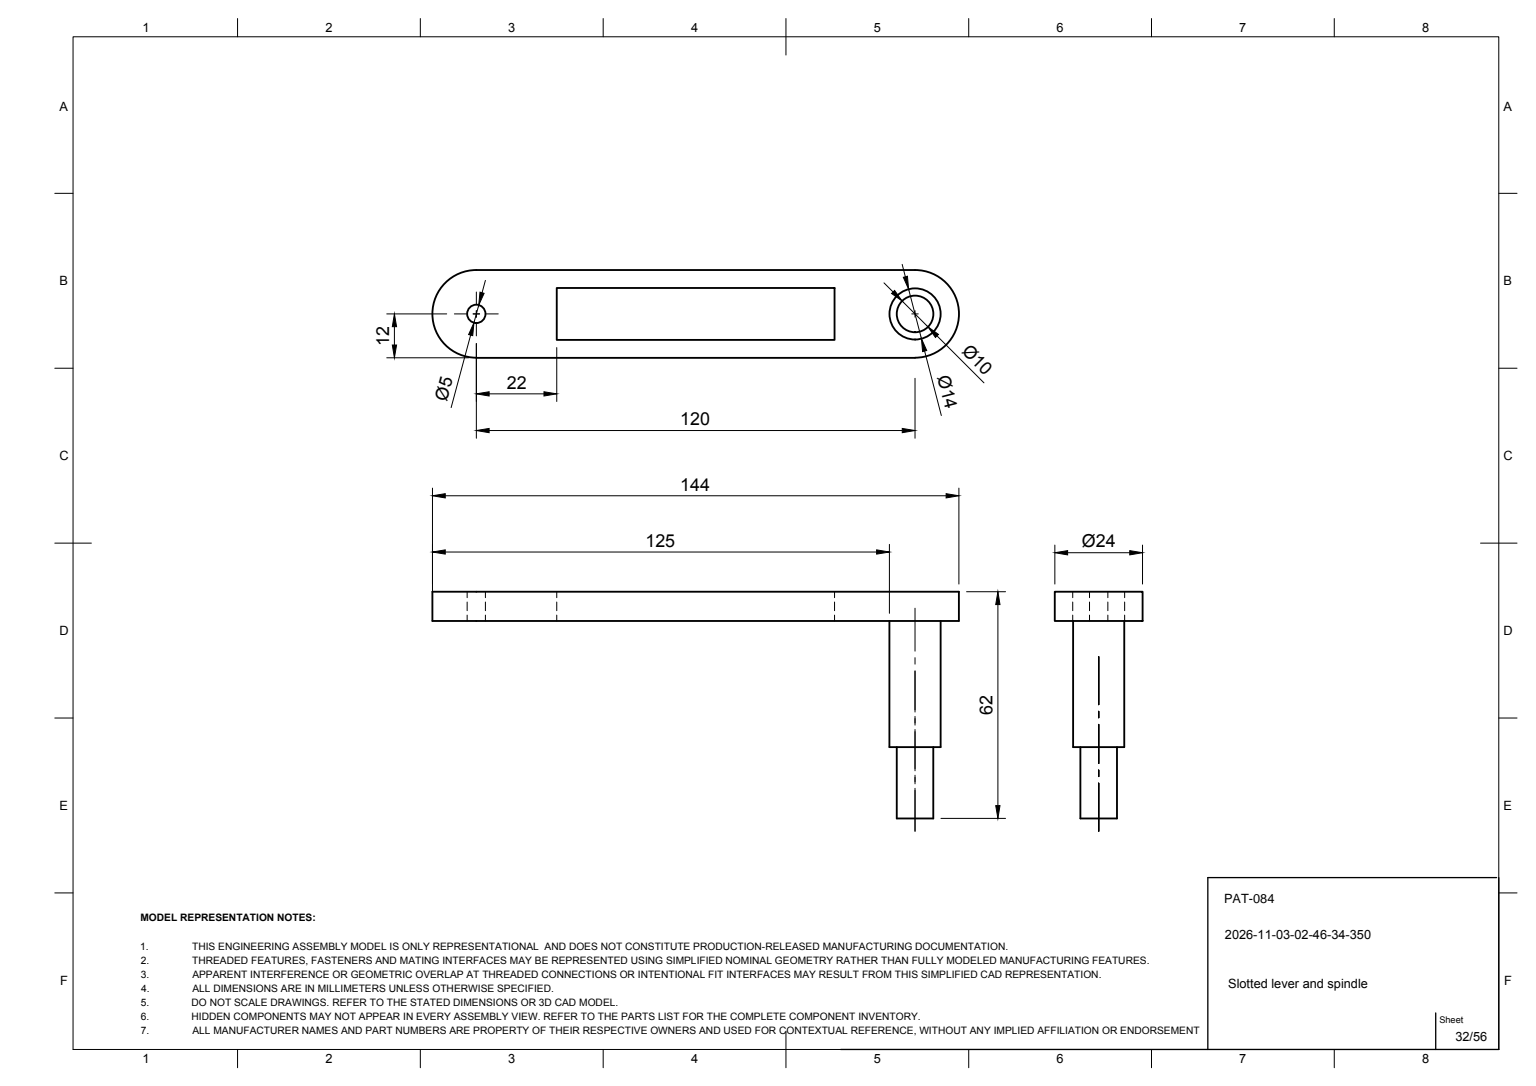
ISO-10303-21;
HEADER;
/* Generated by software containing ST-Developer
 * from STEP Tools, Inc. (www.steptools.com) 
 */

FILE_DESCRIPTION(
/* description */ ('Quick-return (Whitworth) mechanism'),
/* implementation_level */ '2;1');

FILE_NAME(
/* name */ 'Slotted lever and spindle.step',
/* time_stamp */ '2026-10-28T03:25:57-07:00',
/* author */ (''),
/* organization */ (''),
/* preprocessor_version */ 'ST-DEVELOPER v20.2',
/* originating_system */ 'Autodesk Translation Framework v15.17.0.0',
/* authorisation */ '');

FILE_SCHEMA (('AUTOMOTIVE_DESIGN { 1 0 10303 214 3 1 1 }'));
ENDSEC;

DATA;
#10=MECHANICAL_DESIGN_GEOMETRIC_PRESENTATION_REPRESENTATION('',(#520),#14878);
#424=SHAPE_REPRESENTATION_RELATIONSHIP('SRR','None',#15095,#468);
#468=ADVANCED_BREP_SHAPE_REPRESENTATION('',(#571),#14852);
#520=STYLED_ITEM('',(#15399),#571);
#571=MANIFOLD_SOLID_BREP('Body1',#7875);
#725=FACE_BOUND('',#1925,.T.);
#726=FACE_BOUND('',#1926,.T.);
#727=FACE_BOUND('',#1927,.T.);
#728=FACE_BOUND('',#1932,.T.);
#729=FACE_BOUND('',#1936,.T.);
#730=FACE_BOUND('',#1937,.T.);
#912=PLANE('',#8985);
#913=PLANE('',#8986);
#914=PLANE('',#8987);
#915=PLANE('',#8988);
#916=PLANE('',#8992);
#917=PLANE('',#8995);
#918=PLANE('',#8996);
#919=PLANE('',#8999);
#920=PLANE('',#9005);
#921=PLANE('',#9006);
#1318=FACE_OUTER_BOUND('',#1918,.T.);
#1319=FACE_OUTER_BOUND('',#1919,.T.);
#1320=FACE_OUTER_BOUND('',#1920,.T.);
#1321=FACE_OUTER_BOUND('',#1921,.T.);
#1322=FACE_OUTER_BOUND('',#1922,.T.);
#1323=FACE_OUTER_BOUND('',#1923,.T.);
#1324=FACE_OUTER_BOUND('',#1924,.T.);
#1325=FACE_OUTER_BOUND('',#1928,.T.);
#1326=FACE_OUTER_BOUND('',#1929,.T.);
#1327=FACE_OUTER_BOUND('',#1930,.T.);
#1328=FACE_OUTER_BOUND('',#1931,.T.);
#1329=FACE_OUTER_BOUND('',#1933,.T.);
#1330=FACE_OUTER_BOUND('',#1934,.T.);
#1331=FACE_OUTER_BOUND('',#1935,.T.);
#1332=FACE_OUTER_BOUND('',#1938,.T.);
#1918=EDGE_LOOP('',(#6382,#6383,#6384,#6385));
#1919=EDGE_LOOP('',(#6386,#6387,#6388,#6389));
#1920=EDGE_LOOP('',(#6390,#6391,#6392,#6393));
#1921=EDGE_LOOP('',(#6394,#6395,#6396,#6397));
#1922=EDGE_LOOP('',(#6398,#6399,#6400,#6401));
#1923=EDGE_LOOP('',(#6402,#6403,#6404,#6405));
#1924=EDGE_LOOP('',(#6406,#6407,#6408,#6409));
#1925=EDGE_LOOP('',(#6410));
#1926=EDGE_LOOP('',(#6411,#6412,#6413,#6414));
#1927=EDGE_LOOP('',(#6415));
#1928=EDGE_LOOP('',(#6416,#6417,#6418,#6419));
#1929=EDGE_LOOP('',(#6420,#6421,#6422,#6423));
#1930=EDGE_LOOP('',(#6424,#6425,#6426,#6427));
#1931=EDGE_LOOP('',(#6428));
#1932=EDGE_LOOP('',(#6429));
#1933=EDGE_LOOP('',(#6430,#6431,#6432,#6433));
#1934=EDGE_LOOP('',(#6434,#6435,#6436,#6437));
#1935=EDGE_LOOP('',(#6438,#6439,#6440,#6441));
#1936=EDGE_LOOP('',(#6442));
#1937=EDGE_LOOP('',(#6443,#6444,#6445,#6446));
#1938=EDGE_LOOP('',(#6447));
#2405=LINE('',#13732,#2928);
#2406=LINE('',#13737,#2929);
#2407=LINE('',#13739,#2930);
#2408=LINE('',#13741,#2931);
#2409=LINE('',#13742,#2932);
#2410=LINE('',#13745,#2933);
#2411=LINE('',#13747,#2934);
#2412=LINE('',#13748,#2935);
#2413=LINE('',#13751,#2936);
#2414=LINE('',#13753,#2937);
#2415=LINE('',#13754,#2938);
#2416=LINE('',#13756,#2939);
#2417=LINE('',#13757,#2940);
#2418=LINE('',#13761,#2941);
#2419=LINE('',#13765,#2942);
#2420=LINE('',#13769,#2943);
#2421=LINE('',#13772,#2944);
#2422=LINE('',#13777,#2945);
#2423=LINE('',#13778,#2946);
#2424=LINE('',#13781,#2947);
#2425=LINE('',#13782,#2948);
#2426=LINE('',#13791,#2949);
#2427=LINE('',#13794,#2950);
#2928=VECTOR('',#10832,0.25);
#2929=VECTOR('',#10837,1.);
#2930=VECTOR('',#10838,1.);
#2931=VECTOR('',#10839,1.);
#2932=VECTOR('',#10840,1.);
#2933=VECTOR('',#10843,1.);
#2934=VECTOR('',#10844,1.);
#2935=VECTOR('',#10845,1.);
#2936=VECTOR('',#10848,1.);
#2937=VECTOR('',#10849,1.);
#2938=VECTOR('',#10850,1.);
#2939=VECTOR('',#10853,1.);
#2940=VECTOR('',#10854,1.);
#2941=VECTOR('',#10857,1.);
#2942=VECTOR('',#10860,1.);
#2943=VECTOR('',#10865,1.);
#2944=VECTOR('',#10868,1.);
#2945=VECTOR('',#10873,1.);
#2946=VECTOR('',#10874,1.);
#2947=VECTOR('',#10877,1.);
#2948=VECTOR('',#10878,1.);
#2949=VECTOR('',#10891,0.7);
#2950=VECTOR('',#10894,0.5);
#3510=CIRCLE('',#8983,0.25);
#3511=CIRCLE('',#8984,0.25);
#3512=CIRCLE('',#8990,1.2);
#3513=CIRCLE('',#8991,1.2);
#3514=CIRCLE('',#8993,1.2);
#3515=CIRCLE('',#8994,0.7);
#3516=CIRCLE('',#8998,1.2);
#3517=CIRCLE('',#9000,0.7);
#3518=CIRCLE('',#9001,0.5);
#3519=CIRCLE('',#9004,0.5);
#4014=VERTEX_POINT('',#13729);
#4015=VERTEX_POINT('',#13731);
#4016=VERTEX_POINT('',#13735);
#4017=VERTEX_POINT('',#13736);
#4018=VERTEX_POINT('',#13738);
#4019=VERTEX_POINT('',#13740);
#4020=VERTEX_POINT('',#13744);
#4021=VERTEX_POINT('',#13746);
#4022=VERTEX_POINT('',#13750);
#4023=VERTEX_POINT('',#13752);
#4024=VERTEX_POINT('',#13759);
#4025=VERTEX_POINT('',#13760);
#4026=VERTEX_POINT('',#13762);
#4027=VERTEX_POINT('',#13764);
#4028=VERTEX_POINT('',#13768);
#4029=VERTEX_POINT('',#13770);
#4030=VERTEX_POINT('',#13773);
#4031=VERTEX_POINT('',#13776);
#4032=VERTEX_POINT('',#13780);
#4033=VERTEX_POINT('',#13786);
#4034=VERTEX_POINT('',#13788);
#4035=VERTEX_POINT('',#13793);
#4848=EDGE_CURVE('',#4014,#4014,#3510,.T.);
#4849=EDGE_CURVE('',#4014,#4015,#2405,.T.);
#4850=EDGE_CURVE('',#4015,#4015,#3511,.T.);
#4851=EDGE_CURVE('',#4016,#4017,#2406,.T.);
#4852=EDGE_CURVE('',#4016,#4018,#2407,.T.);
#4853=EDGE_CURVE('',#4019,#4018,#2408,.T.);
#4854=EDGE_CURVE('',#4017,#4019,#2409,.T.);
#4855=EDGE_CURVE('',#4017,#4020,#2410,.T.);
#4856=EDGE_CURVE('',#4021,#4019,#2411,.T.);
#4857=EDGE_CURVE('',#4020,#4021,#2412,.T.);
#4858=EDGE_CURVE('',#4020,#4022,#2413,.T.);
#4859=EDGE_CURVE('',#4023,#4021,#2414,.T.);
#4860=EDGE_CURVE('',#4022,#4023,#2415,.T.);
#4861=EDGE_CURVE('',#4022,#4016,#2416,.T.);
#4862=EDGE_CURVE('',#4018,#4023,#2417,.T.);
#4863=EDGE_CURVE('',#4024,#4025,#2418,.T.);
#4864=EDGE_CURVE('',#4026,#4025,#3512,.T.);
#4865=EDGE_CURVE('',#4027,#4026,#2419,.T.);
#4866=EDGE_CURVE('',#4027,#4024,#3513,.T.);
#4867=EDGE_CURVE('',#4027,#4028,#2420,.T.);
#4868=EDGE_CURVE('',#4029,#4028,#3514,.T.);
#4869=EDGE_CURVE('',#4029,#4024,#2421,.T.);
#4870=EDGE_CURVE('',#4030,#4030,#3515,.T.);
#4871=EDGE_CURVE('',#4031,#4029,#2422,.T.);
#4872=EDGE_CURVE('',#4025,#4031,#2423,.T.);
#4873=EDGE_CURVE('',#4032,#4026,#2424,.T.);
#4874=EDGE_CURVE('',#4028,#4032,#2425,.T.);
#4875=EDGE_CURVE('',#4031,#4032,#3516,.T.);
#4876=EDGE_CURVE('',#4033,#4033,#3517,.T.);
#4877=EDGE_CURVE('',#4034,#4034,#3518,.T.);
#4878=EDGE_CURVE('',#4030,#4033,#2426,.T.);
#4879=EDGE_CURVE('',#4034,#4035,#2427,.T.);
#4880=EDGE_CURVE('',#4035,#4035,#3519,.T.);
#6382=ORIENTED_EDGE('',*,*,#4848,.F.);
#6383=ORIENTED_EDGE('',*,*,#4849,.T.);
#6384=ORIENTED_EDGE('',*,*,#4850,.F.);
#6385=ORIENTED_EDGE('',*,*,#4849,.F.);
#6386=ORIENTED_EDGE('',*,*,#4851,.F.);
#6387=ORIENTED_EDGE('',*,*,#4852,.T.);
#6388=ORIENTED_EDGE('',*,*,#4853,.F.);
#6389=ORIENTED_EDGE('',*,*,#4854,.F.);
#6390=ORIENTED_EDGE('',*,*,#4855,.F.);
#6391=ORIENTED_EDGE('',*,*,#4854,.T.);
#6392=ORIENTED_EDGE('',*,*,#4856,.F.);
#6393=ORIENTED_EDGE('',*,*,#4857,.F.);
#6394=ORIENTED_EDGE('',*,*,#4858,.F.);
#6395=ORIENTED_EDGE('',*,*,#4857,.T.);
#6396=ORIENTED_EDGE('',*,*,#4859,.F.);
#6397=ORIENTED_EDGE('',*,*,#4860,.F.);
#6398=ORIENTED_EDGE('',*,*,#4861,.F.);
#6399=ORIENTED_EDGE('',*,*,#4860,.T.);
#6400=ORIENTED_EDGE('',*,*,#4862,.F.);
#6401=ORIENTED_EDGE('',*,*,#4852,.F.);
#6402=ORIENTED_EDGE('',*,*,#4863,.T.);
#6403=ORIENTED_EDGE('',*,*,#4864,.F.);
#6404=ORIENTED_EDGE('',*,*,#4865,.F.);
#6405=ORIENTED_EDGE('',*,*,#4866,.T.);
#6406=ORIENTED_EDGE('',*,*,#4867,.T.);
#6407=ORIENTED_EDGE('',*,*,#4868,.F.);
#6408=ORIENTED_EDGE('',*,*,#4869,.T.);
#6409=ORIENTED_EDGE('',*,*,#4866,.F.);
#6410=ORIENTED_EDGE('',*,*,#4848,.T.);
#6411=ORIENTED_EDGE('',*,*,#4858,.T.);
#6412=ORIENTED_EDGE('',*,*,#4861,.T.);
#6413=ORIENTED_EDGE('',*,*,#4851,.T.);
#6414=ORIENTED_EDGE('',*,*,#4855,.T.);
#6415=ORIENTED_EDGE('',*,*,#4870,.T.);
#6416=ORIENTED_EDGE('',*,*,#4869,.F.);
#6417=ORIENTED_EDGE('',*,*,#4871,.F.);
#6418=ORIENTED_EDGE('',*,*,#4872,.F.);
#6419=ORIENTED_EDGE('',*,*,#4863,.F.);
#6420=ORIENTED_EDGE('',*,*,#4867,.F.);
#6421=ORIENTED_EDGE('',*,*,#4865,.T.);
#6422=ORIENTED_EDGE('',*,*,#4873,.F.);
#6423=ORIENTED_EDGE('',*,*,#4874,.F.);
#6424=ORIENTED_EDGE('',*,*,#4871,.T.);
#6425=ORIENTED_EDGE('',*,*,#4868,.T.);
#6426=ORIENTED_EDGE('',*,*,#4874,.T.);
#6427=ORIENTED_EDGE('',*,*,#4875,.F.);
#6428=ORIENTED_EDGE('',*,*,#4876,.F.);
#6429=ORIENTED_EDGE('',*,*,#4877,.F.);
#6430=ORIENTED_EDGE('',*,*,#4870,.F.);
#6431=ORIENTED_EDGE('',*,*,#4878,.T.);
#6432=ORIENTED_EDGE('',*,*,#4876,.T.);
#6433=ORIENTED_EDGE('',*,*,#4878,.F.);
#6434=ORIENTED_EDGE('',*,*,#4877,.T.);
#6435=ORIENTED_EDGE('',*,*,#4879,.T.);
#6436=ORIENTED_EDGE('',*,*,#4880,.T.);
#6437=ORIENTED_EDGE('',*,*,#4879,.F.);
#6438=ORIENTED_EDGE('',*,*,#4872,.T.);
#6439=ORIENTED_EDGE('',*,*,#4875,.T.);
#6440=ORIENTED_EDGE('',*,*,#4873,.T.);
#6441=ORIENTED_EDGE('',*,*,#4864,.T.);
#6442=ORIENTED_EDGE('',*,*,#4850,.T.);
#6443=ORIENTED_EDGE('',*,*,#4859,.T.);
#6444=ORIENTED_EDGE('',*,*,#4856,.T.);
#6445=ORIENTED_EDGE('',*,*,#4853,.T.);
#6446=ORIENTED_EDGE('',*,*,#4862,.T.);
#6447=ORIENTED_EDGE('',*,*,#4880,.F.);
#7325=CYLINDRICAL_SURFACE('',#8982,0.25);
#7326=CYLINDRICAL_SURFACE('',#8989,1.2);
#7327=CYLINDRICAL_SURFACE('',#8997,1.2);
#7328=CYLINDRICAL_SURFACE('',#9002,0.7);
#7329=CYLINDRICAL_SURFACE('',#9003,0.5);
#7649=ADVANCED_FACE('',(#1318),#7325,.F.);
#7650=ADVANCED_FACE('',(#1319),#912,.F.);
#7651=ADVANCED_FACE('',(#1320),#913,.F.);
#7652=ADVANCED_FACE('',(#1321),#914,.F.);
#7653=ADVANCED_FACE('',(#1322),#915,.F.);
#7654=ADVANCED_FACE('',(#1323),#7326,.T.);
#7655=ADVANCED_FACE('',(#1324,#725,#726,#727),#916,.F.);
#7656=ADVANCED_FACE('',(#1325),#917,.T.);
#7657=ADVANCED_FACE('',(#1326),#918,.T.);
#7658=ADVANCED_FACE('',(#1327),#7327,.T.);
#7659=ADVANCED_FACE('',(#1328,#728),#919,.F.);
#7660=ADVANCED_FACE('',(#1329),#7328,.T.);
#7661=ADVANCED_FACE('',(#1330),#7329,.T.);
#7662=ADVANCED_FACE('',(#1331,#729,#730),#920,.T.);
#7663=ADVANCED_FACE('',(#1332),#921,.F.);
#7875=CLOSED_SHELL('',(#7649,#7650,#7651,#7652,#7653,#7654,#7655,#7656,
#7657,#7658,#7659,#7660,#7661,#7662,#7663));
#8981=AXIS2_PLACEMENT_3D('',#13727,#10826,#10827);
#8982=AXIS2_PLACEMENT_3D('',#13728,#10828,#10829);
#8983=AXIS2_PLACEMENT_3D('',#13730,#10830,#10831);
#8984=AXIS2_PLACEMENT_3D('',#13733,#10833,#10834);
#8985=AXIS2_PLACEMENT_3D('',#13734,#10835,#10836);
#8986=AXIS2_PLACEMENT_3D('',#13743,#10841,#10842);
#8987=AXIS2_PLACEMENT_3D('',#13749,#10846,#10847);
#8988=AXIS2_PLACEMENT_3D('',#13755,#10851,#10852);
#8989=AXIS2_PLACEMENT_3D('',#13758,#10855,#10856);
#8990=AXIS2_PLACEMENT_3D('',#13763,#10858,#10859);
#8991=AXIS2_PLACEMENT_3D('',#13766,#10861,#10862);
#8992=AXIS2_PLACEMENT_3D('',#13767,#10863,#10864);
#8993=AXIS2_PLACEMENT_3D('',#13771,#10866,#10867);
#8994=AXIS2_PLACEMENT_3D('',#13774,#10869,#10870);
#8995=AXIS2_PLACEMENT_3D('',#13775,#10871,#10872);
#8996=AXIS2_PLACEMENT_3D('',#13779,#10875,#10876);
#8997=AXIS2_PLACEMENT_3D('',#13783,#10879,#10880);
#8998=AXIS2_PLACEMENT_3D('',#13784,#10881,#10882);
#8999=AXIS2_PLACEMENT_3D('',#13785,#10883,#10884);
#9000=AXIS2_PLACEMENT_3D('',#13787,#10885,#10886);
#9001=AXIS2_PLACEMENT_3D('',#13789,#10887,#10888);
#9002=AXIS2_PLACEMENT_3D('',#13790,#10889,#10890);
#9003=AXIS2_PLACEMENT_3D('',#13792,#10892,#10893);
#9004=AXIS2_PLACEMENT_3D('',#13795,#10895,#10896);
#9005=AXIS2_PLACEMENT_3D('',#13796,#10897,#10898);
#9006=AXIS2_PLACEMENT_3D('',#13797,#10899,#10900);
#10826=DIRECTION('axis',(0.,0.,1.));
#10827=DIRECTION('refdir',(1.,0.,0.));
#10828=DIRECTION('center_axis',(0.,0.,1.));
#10829=DIRECTION('ref_axis',(1.,0.,0.));
#10830=DIRECTION('center_axis',(0.,0.,1.));
#10831=DIRECTION('ref_axis',(1.,0.,0.));
#10832=DIRECTION('',(0.,0.,1.));
#10833=DIRECTION('center_axis',(0.,0.,-1.));
#10834=DIRECTION('ref_axis',(1.,0.,0.));
#10835=DIRECTION('center_axis',(0.,-1.,0.));
#10836=DIRECTION('ref_axis',(1.,0.,0.));
#10837=DIRECTION('',(1.,0.,0.));
#10838=DIRECTION('',(0.,0.,1.));
#10839=DIRECTION('',(-1.,0.,0.));
#10840=DIRECTION('',(0.,0.,1.));
#10841=DIRECTION('center_axis',(1.,0.,0.));
#10842=DIRECTION('ref_axis',(0.,1.,0.));
#10843=DIRECTION('',(0.,1.,0.));
#10844=DIRECTION('',(0.,-1.,0.));
#10845=DIRECTION('',(0.,0.,1.));
#10846=DIRECTION('center_axis',(0.,1.,0.));
#10847=DIRECTION('ref_axis',(-1.,0.,0.));
#10848=DIRECTION('',(-1.,0.,0.));
#10849=DIRECTION('',(1.,0.,0.));
#10850=DIRECTION('',(0.,0.,1.));
#10851=DIRECTION('center_axis',(-1.,0.,0.));
#10852=DIRECTION('ref_axis',(0.,-1.,0.));
#10853=DIRECTION('',(0.,-1.,0.));
#10854=DIRECTION('',(0.,1.,0.));
#10855=DIRECTION('center_axis',(0.,0.,1.));
#10856=DIRECTION('ref_axis',(1.,0.,0.));
#10857=DIRECTION('',(0.,0.,1.));
#10858=DIRECTION('center_axis',(0.,0.,1.));
#10859=DIRECTION('ref_axis',(1.,0.,0.));
#10860=DIRECTION('',(0.,0.,1.));
#10861=DIRECTION('center_axis',(0.,0.,1.));
#10862=DIRECTION('ref_axis',(1.,0.,0.));
#10863=DIRECTION('center_axis',(0.,0.,1.));
#10864=DIRECTION('ref_axis',(1.,0.,0.));
#10865=DIRECTION('',(0.,-1.,0.));
#10866=DIRECTION('center_axis',(0.,0.,1.));
#10867=DIRECTION('ref_axis',(1.,0.,0.));
#10868=DIRECTION('',(0.,1.,0.));
#10869=DIRECTION('center_axis',(0.,0.,1.));
#10870=DIRECTION('ref_axis',(1.,0.,0.));
#10871=DIRECTION('center_axis',(-1.,0.,0.));
#10872=DIRECTION('ref_axis',(0.,-1.,0.));
#10873=DIRECTION('',(0.,0.,-1.));
#10874=DIRECTION('',(0.,-1.,0.));
#10875=DIRECTION('center_axis',(1.,0.,0.));
#10876=DIRECTION('ref_axis',(0.,1.,0.));
#10877=DIRECTION('',(0.,1.,0.));
#10878=DIRECTION('',(0.,0.,1.));
#10879=DIRECTION('center_axis',(0.,0.,1.));
#10880=DIRECTION('ref_axis',(1.,0.,0.));
#10881=DIRECTION('center_axis',(0.,0.,1.));
#10882=DIRECTION('ref_axis',(1.,0.,0.));
#10883=DIRECTION('center_axis',(0.,0.,1.));
#10884=DIRECTION('ref_axis',(1.,0.,0.));
#10885=DIRECTION('center_axis',(0.,0.,1.));
#10886=DIRECTION('ref_axis',(1.,0.,0.));
#10887=DIRECTION('center_axis',(0.,0.,-1.));
#10888=DIRECTION('ref_axis',(1.,0.,0.));
#10889=DIRECTION('center_axis',(0.,0.,1.));
#10890=DIRECTION('ref_axis',(1.,0.,0.));
#10891=DIRECTION('',(0.,0.,-1.));
#10892=DIRECTION('center_axis',(0.,0.,1.));
#10893=DIRECTION('ref_axis',(1.,0.,0.));
#10894=DIRECTION('',(0.,0.,-1.));
#10895=DIRECTION('center_axis',(0.,0.,1.));
#10896=DIRECTION('ref_axis',(1.,0.,0.));
#10897=DIRECTION('center_axis',(0.,0.,1.));
#10898=DIRECTION('ref_axis',(1.,0.,0.));
#10899=DIRECTION('center_axis',(0.,0.,1.));
#10900=DIRECTION('ref_axis',(1.,0.,0.));
#13727=CARTESIAN_POINT('',(0.,0.,0.));
#13728=CARTESIAN_POINT('Origin',(0.,12.,6.3));
#13729=CARTESIAN_POINT('',(-0.25,12.,6.4));
#13730=CARTESIAN_POINT('Origin',(0.,12.,6.4));
#13731=CARTESIAN_POINT('',(-0.25,12.,7.2));
#13732=CARTESIAN_POINT('',(-0.25,12.,6.3));
#13733=CARTESIAN_POINT('Origin',(0.,12.,7.2));
#13734=CARTESIAN_POINT('Origin',(-0.71,2.2,6.3));
#13735=CARTESIAN_POINT('',(-0.71,2.2,6.4));
#13736=CARTESIAN_POINT('',(0.71,2.2,6.4));
#13737=CARTESIAN_POINT('',(-0.355,2.2,6.4));
#13738=CARTESIAN_POINT('',(-0.71,2.2,7.2));
#13739=CARTESIAN_POINT('',(-0.71,2.2,6.3));
#13740=CARTESIAN_POINT('',(0.71,2.2,7.2));
#13741=CARTESIAN_POINT('',(-0.355,2.2,7.2));
#13742=CARTESIAN_POINT('',(0.71,2.2,6.3));
#13743=CARTESIAN_POINT('Origin',(0.71,2.2,6.3));
#13744=CARTESIAN_POINT('',(0.71,9.8,6.4));
#13745=CARTESIAN_POINT('',(0.71,1.1,6.4));
#13746=CARTESIAN_POINT('',(0.71,9.8,7.2));
#13747=CARTESIAN_POINT('',(0.71,1.1,7.2));
#13748=CARTESIAN_POINT('',(0.71,9.8,6.3));
#13749=CARTESIAN_POINT('Origin',(0.71,9.8,6.3));
#13750=CARTESIAN_POINT('',(-0.71,9.8,6.4));
#13751=CARTESIAN_POINT('',(0.355,9.8,6.4));
#13752=CARTESIAN_POINT('',(-0.71,9.8,7.2));
#13753=CARTESIAN_POINT('',(0.355,9.8,7.2));
#13754=CARTESIAN_POINT('',(-0.71,9.8,6.3));
#13755=CARTESIAN_POINT('Origin',(-0.71,9.8,6.3));
#13756=CARTESIAN_POINT('',(-0.71,4.9,6.4));
#13757=CARTESIAN_POINT('',(-0.71,4.9,7.2));
#13758=CARTESIAN_POINT('Origin',(0.,12.,6.4));
#13759=CARTESIAN_POINT('',(-1.2,12.,6.4));
#13760=CARTESIAN_POINT('',(-1.2,12.,7.2));
#13761=CARTESIAN_POINT('',(-1.2,12.,6.4));
#13762=CARTESIAN_POINT('',(1.2,12.,7.2));
#13763=CARTESIAN_POINT('Origin',(0.,12.,7.2));
#13764=CARTESIAN_POINT('',(1.2,12.,6.4));
#13765=CARTESIAN_POINT('',(1.2,12.,6.4));
#13766=CARTESIAN_POINT('Origin',(0.,12.,6.4));
#13767=CARTESIAN_POINT('Origin',(0.,0.,6.4));
#13768=CARTESIAN_POINT('',(1.2,0.,6.4));
#13769=CARTESIAN_POINT('',(1.2,12.,6.4));
#13770=CARTESIAN_POINT('',(-1.2,-1.46957615897682E-16,6.4));
#13771=CARTESIAN_POINT('Origin',(0.,0.,6.4));
#13772=CARTESIAN_POINT('',(-1.2,0.,6.4));
#13773=CARTESIAN_POINT('',(-0.7,-8.57252759403147E-17,6.4));
#13774=CARTESIAN_POINT('Origin',(0.,0.,6.4));
#13775=CARTESIAN_POINT('Origin',(-1.2,12.,6.4));
#13776=CARTESIAN_POINT('',(-1.2,-1.46957615897682E-16,7.2));
#13777=CARTESIAN_POINT('',(-1.2,0.,6.4));
#13778=CARTESIAN_POINT('',(-1.2,0.,7.2));
#13779=CARTESIAN_POINT('Origin',(1.2,0.,6.4));
#13780=CARTESIAN_POINT('',(1.2,0.,7.2));
#13781=CARTESIAN_POINT('',(1.2,12.,7.2));
#13782=CARTESIAN_POINT('',(1.2,0.,6.4));
#13783=CARTESIAN_POINT('Origin',(0.,0.,6.4));
#13784=CARTESIAN_POINT('Origin',(0.,0.,7.2));
#13785=CARTESIAN_POINT('Origin',(0.,0.,2.95));
#13786=CARTESIAN_POINT('',(-0.7,-8.57252759403147E-17,2.95));
#13787=CARTESIAN_POINT('Origin',(0.,0.,2.95));
#13788=CARTESIAN_POINT('',(-0.5,6.12323399573677E-17,2.95));
#13789=CARTESIAN_POINT('Origin',(0.,0.,2.95));
#13790=CARTESIAN_POINT('Origin',(0.,0.,2.95));
#13791=CARTESIAN_POINT('',(-0.7,-8.57252759403147E-17,2.95));
#13792=CARTESIAN_POINT('Origin',(0.,0.,1.));
#13793=CARTESIAN_POINT('',(-0.5,-6.12323399573677E-17,1.));
#13794=CARTESIAN_POINT('',(-0.5,-6.12323399573677E-17,1.));
#13795=CARTESIAN_POINT('Origin',(0.,0.,1.));
#13796=CARTESIAN_POINT('Origin',(0.,0.,7.2));
#13797=CARTESIAN_POINT('Origin',(0.,0.,1.));
#14798=UNCERTAINTY_MEASURE_WITH_UNIT(LENGTH_MEASURE(0.001),#14879,
'DISTANCE_ACCURACY_VALUE',
'Maximum model space distance between geometric entities at asserted c
onnectivities');
#14824=UNCERTAINTY_MEASURE_WITH_UNIT(LENGTH_MEASURE(0.001),#14879,
'DISTANCE_ACCURACY_VALUE',
'Maximum model space distance between geometric entities at asserted c
onnectivities');
#14852=(
GEOMETRIC_REPRESENTATION_CONTEXT(3)
GLOBAL_UNCERTAINTY_ASSIGNED_CONTEXT((#14798))
GLOBAL_UNIT_ASSIGNED_CONTEXT((#14879,#14881,#14882))
REPRESENTATION_CONTEXT('','3D')
);
#14878=(
GEOMETRIC_REPRESENTATION_CONTEXT(3)
GLOBAL_UNCERTAINTY_ASSIGNED_CONTEXT((#14824))
GLOBAL_UNIT_ASSIGNED_CONTEXT((#14879,#14881,#14882))
REPRESENTATION_CONTEXT('','3D')
);
#14879=(
LENGTH_UNIT()
NAMED_UNIT(*)
SI_UNIT(.CENTI.,.METRE.)
);
#14881=(
NAMED_UNIT(*)
PLANE_ANGLE_UNIT()
SI_UNIT($,.RADIAN.)
);
#14882=(
NAMED_UNIT(*)
SI_UNIT($,.STERADIAN.)
SOLID_ANGLE_UNIT()
);
#14910=SHAPE_DEFINITION_REPRESENTATION(#14968,#15095);
#14968=PRODUCT_DEFINITION_SHAPE('',$,#15149);
#15095=SHAPE_REPRESENTATION('',(#8981),#14852);
#15121=PRODUCT_DEFINITION_CONTEXT('part definition',#15282,'design');
#15149=PRODUCT_DEFINITION('Slotted lever and spindle',
'Slotted lever and spindle',#15202,#15121);
#15202=PRODUCT_DEFINITION_FORMATION('',$,#15311);
#15282=APPLICATION_CONTEXT(
'Core Data for Automotive Mechanical Design Process');
#15283=PRODUCT_CONTEXT('part definition',#15282,'mechanical');
#15311=PRODUCT('Slotted lever and spindle','Slotted lever and spindle',
'Slotted lever and spindle',(#15283));
#15393=COLOUR_RGB('Sky Blue',0.24,0.69,0.87);
#15394=FILL_AREA_STYLE_COLOUR('',#15393);
#15395=FILL_AREA_STYLE('',(#15394));
#15396=SURFACE_STYLE_FILL_AREA(#15395);
#15397=SURFACE_SIDE_STYLE('',(#15396));
#15398=SURFACE_STYLE_USAGE(.BOTH.,#15397);
#15399=PRESENTATION_STYLE_ASSIGNMENT((#15398));
ENDSEC;
END-ISO-10303-21;
